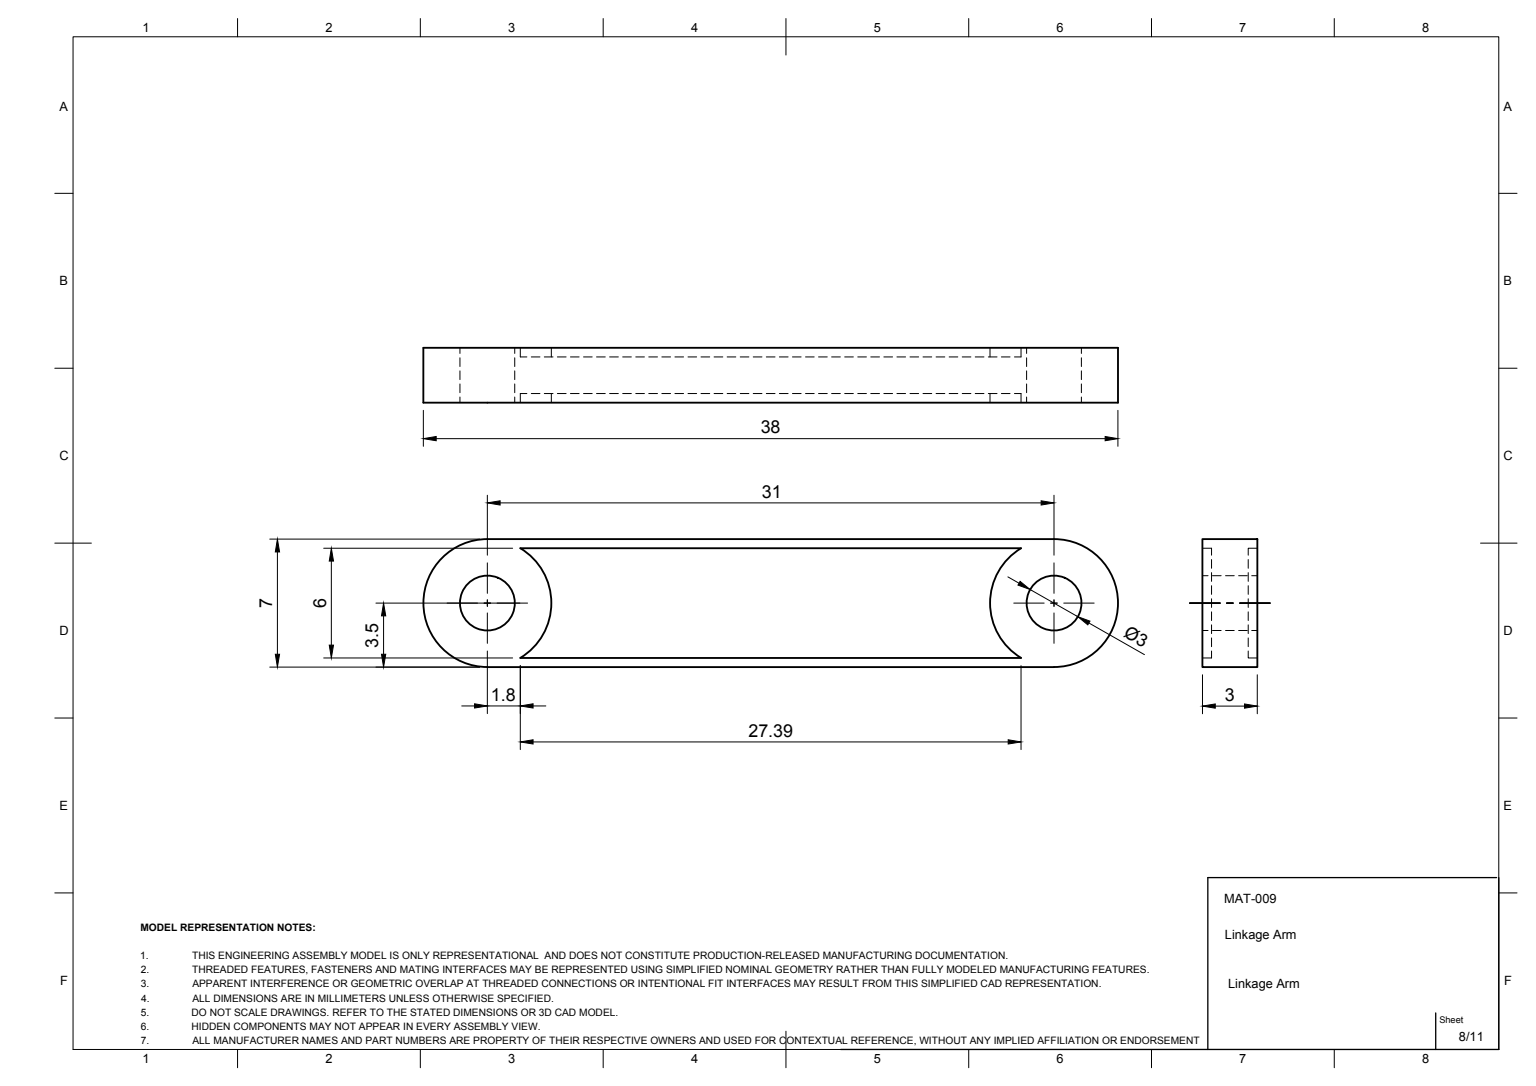
ISO-10303-21;
HEADER;
/* Generated by software containing ST-Developer
 * from STEP Tools, Inc. (www.steptools.com) 
 */

FILE_DESCRIPTION(
/* description */ ('STEP AP214'),
/* implementation_level */ '2;1');

FILE_NAME(
/* name */ 'Linkage Arm.step',
/* time_stamp */ '2026-11-14T05:43:09-08:00',
/* author */ (''),
/* organization */ (''),
/* preprocessor_version */ 'ST-DEVELOPER v20.2',
/* originating_system */ 'Autodesk Translation Framework v15.17.0.0',
/* authorisation */ '');

FILE_SCHEMA (('AUTOMOTIVE_DESIGN { 1 0 10303 214 3 1 1 }'));
ENDSEC;

DATA;
#10=MECHANICAL_DESIGN_GEOMETRIC_PRESENTATION_REPRESENTATION('',(#152),#11933);
#134=SHAPE_REPRESENTATION_RELATIONSHIP('SRR','None',#11994,#143);
#143=ADVANCED_BREP_SHAPE_REPRESENTATION('',(#161),#11930);
#152=STYLED_ITEM('',(#12044),#161);
#161=MANIFOLD_SOLID_BREP('Body1',#6649);
#200=FACE_BOUND('',#1019,.T.);
#201=FACE_BOUND('',#1020,.T.);
#202=FACE_BOUND('',#1021,.T.);
#203=FACE_BOUND('',#1026,.T.);
#204=FACE_BOUND('',#1027,.T.);
#205=FACE_BOUND('',#1028,.T.);
#288=PLANE('',#7537);
#289=PLANE('',#7540);
#290=PLANE('',#7541);
#291=PLANE('',#7544);
#292=PLANE('',#7546);
#293=PLANE('',#7549);
#294=PLANE('',#7550);
#295=PLANE('',#7553);
#296=PLANE('',#7554);
#297=PLANE('',#7555);
#623=FACE_OUTER_BOUND('',#1013,.T.);
#624=FACE_OUTER_BOUND('',#1014,.T.);
#625=FACE_OUTER_BOUND('',#1015,.T.);
#626=FACE_OUTER_BOUND('',#1016,.T.);
#627=FACE_OUTER_BOUND('',#1017,.T.);
#628=FACE_OUTER_BOUND('',#1018,.T.);
#629=FACE_OUTER_BOUND('',#1022,.T.);
#630=FACE_OUTER_BOUND('',#1023,.T.);
#631=FACE_OUTER_BOUND('',#1024,.T.);
#632=FACE_OUTER_BOUND('',#1025,.T.);
#633=FACE_OUTER_BOUND('',#1029,.T.);
#634=FACE_OUTER_BOUND('',#1030,.T.);
#635=FACE_OUTER_BOUND('',#1031,.T.);
#636=FACE_OUTER_BOUND('',#1032,.T.);
#637=FACE_OUTER_BOUND('',#1033,.T.);
#638=FACE_OUTER_BOUND('',#1034,.T.);
#639=FACE_OUTER_BOUND('',#1035,.T.);
#640=FACE_OUTER_BOUND('',#1036,.T.);
#1013=EDGE_LOOP('',(#5812,#5813,#5814,#5815));
#1014=EDGE_LOOP('',(#5816,#5817,#5818,#5819));
#1015=EDGE_LOOP('',(#5820,#5821,#5822,#5823));
#1016=EDGE_LOOP('',(#5824,#5825,#5826,#5827));
#1017=EDGE_LOOP('',(#5828,#5829,#5830,#5831));
#1018=EDGE_LOOP('',(#5832,#5833,#5834,#5835));
#1019=EDGE_LOOP('',(#5836));
#1020=EDGE_LOOP('',(#5837));
#1021=EDGE_LOOP('',(#5838,#5839,#5840,#5841));
#1022=EDGE_LOOP('',(#5842,#5843,#5844,#5845));
#1023=EDGE_LOOP('',(#5846,#5847,#5848,#5849));
#1024=EDGE_LOOP('',(#5850,#5851,#5852,#5853));
#1025=EDGE_LOOP('',(#5854,#5855,#5856,#5857));
#1026=EDGE_LOOP('',(#5858,#5859,#5860,#5861));
#1027=EDGE_LOOP('',(#5862));
#1028=EDGE_LOOP('',(#5863));
#1029=EDGE_LOOP('',(#5864,#5865,#5866,#5867));
#1030=EDGE_LOOP('',(#5868,#5869,#5870,#5871));
#1031=EDGE_LOOP('',(#5872,#5873,#5874,#5875));
#1032=EDGE_LOOP('',(#5876,#5877,#5878,#5879));
#1033=EDGE_LOOP('',(#5880,#5881,#5882,#5883));
#1034=EDGE_LOOP('',(#5884,#5885,#5886,#5887));
#1035=EDGE_LOOP('',(#5888,#5889,#5890,#5891));
#1036=EDGE_LOOP('',(#5892,#5893,#5894,#5895));
#1464=LINE('',#11641,#1926);
#1465=LINE('',#11644,#1927);
#1466=LINE('',#11650,#1928);
#1467=LINE('',#11653,#1929);
#1468=LINE('',#11658,#1930);
#1469=LINE('',#11664,#1931);
#1470=LINE('',#11671,#1932);
#1471=LINE('',#11674,#1933);
#1472=LINE('',#11677,#1934);
#1473=LINE('',#11680,#1935);
#1474=LINE('',#11684,#1936);
#1475=LINE('',#11685,#1937);
#1476=LINE('',#11688,#1938);
#1477=LINE('',#11689,#1939);
#1478=LINE('',#11692,#1940);
#1479=LINE('',#11693,#1941);
#1480=LINE('',#11698,#1942);
#1481=LINE('',#11701,#1943);
#1482=LINE('',#11704,#1944);
#1483=LINE('',#11705,#1945);
#1484=LINE('',#11709,#1946);
#1485=LINE('',#11711,#1947);
#1486=LINE('',#11715,#1948);
#1487=LINE('',#11718,#1949);
#1488=LINE('',#11720,#1950);
#1489=LINE('',#11722,#1951);
#1926=VECTOR('',#9586,1000.);
#1927=VECTOR('',#9589,1000.);
#1928=VECTOR('',#9594,1000.);
#1929=VECTOR('',#9597,1000.);
#1930=VECTOR('',#9602,1.5);
#1931=VECTOR('',#9609,1.5);
#1932=VECTOR('',#9616,1000.);
#1933=VECTOR('',#9619,1000.);
#1934=VECTOR('',#9622,1000.);
#1935=VECTOR('',#9625,1000.);
#1936=VECTOR('',#9628,1000.);
#1937=VECTOR('',#9629,1000.);
#1938=VECTOR('',#9632,1000.);
#1939=VECTOR('',#9633,1000.);
#1940=VECTOR('',#9636,1000.);
#1941=VECTOR('',#9637,1000.);
#1942=VECTOR('',#9644,1000.);
#1943=VECTOR('',#9647,1000.);
#1944=VECTOR('',#9650,1000.);
#1945=VECTOR('',#9651,1000.);
#1946=VECTOR('',#9656,1000.);
#1947=VECTOR('',#9659,1000.);
#1948=VECTOR('',#9664,1000.);
#1949=VECTOR('',#9667,1000.);
#1950=VECTOR('',#9670,1000.);
#1951=VECTOR('',#9673,1000.);
#2454=CIRCLE('',#7523,3.5);
#2455=CIRCLE('',#7524,3.5);
#2456=CIRCLE('',#7526,3.5);
#2457=CIRCLE('',#7527,3.5);
#2458=CIRCLE('',#7529,1.5);
#2459=CIRCLE('',#7530,1.5);
#2460=CIRCLE('',#7532,1.5);
#2461=CIRCLE('',#7533,1.5);
#2462=CIRCLE('',#7535,3.5);
#2463=CIRCLE('',#7536,3.5);
#2464=CIRCLE('',#7538,3.5);
#2465=CIRCLE('',#7539,3.5);
#2466=CIRCLE('',#7543,3.5);
#2467=CIRCLE('',#7545,3.5);
#2468=CIRCLE('',#7548,3.5);
#2469=CIRCLE('',#7552,3.5);
#3067=VERTEX_POINT('',#11637);
#3068=VERTEX_POINT('',#11638);
#3069=VERTEX_POINT('',#11640);
#3070=VERTEX_POINT('',#11642);
#3071=VERTEX_POINT('',#11646);
#3072=VERTEX_POINT('',#11647);
#3073=VERTEX_POINT('',#11649);
#3074=VERTEX_POINT('',#11651);
#3075=VERTEX_POINT('',#11655);
#3076=VERTEX_POINT('',#11657);
#3077=VERTEX_POINT('',#11661);
#3078=VERTEX_POINT('',#11663);
#3079=VERTEX_POINT('',#11667);
#3080=VERTEX_POINT('',#11668);
#3081=VERTEX_POINT('',#11670);
#3082=VERTEX_POINT('',#11672);
#3083=VERTEX_POINT('',#11676);
#3084=VERTEX_POINT('',#11678);
#3085=VERTEX_POINT('',#11681);
#3086=VERTEX_POINT('',#11682);
#3087=VERTEX_POINT('',#11687);
#3088=VERTEX_POINT('',#11691);
#3089=VERTEX_POINT('',#11697);
#3090=VERTEX_POINT('',#11699);
#3091=VERTEX_POINT('',#11703);
#3092=VERTEX_POINT('',#11707);
#3093=VERTEX_POINT('',#11714);
#3094=VERTEX_POINT('',#11716);
#3995=EDGE_CURVE('',#3067,#3068,#2454,.T.);
#3996=EDGE_CURVE('',#3068,#3069,#1464,.T.);
#3997=EDGE_CURVE('',#3070,#3069,#2455,.T.);
#3998=EDGE_CURVE('',#3067,#3070,#1465,.T.);
#3999=EDGE_CURVE('',#3071,#3072,#2456,.T.);
#4000=EDGE_CURVE('',#3071,#3073,#1466,.T.);
#4001=EDGE_CURVE('',#3073,#3074,#2457,.T.);
#4002=EDGE_CURVE('',#3072,#3074,#1467,.T.);
#4003=EDGE_CURVE('',#3075,#3075,#2458,.T.);
#4004=EDGE_CURVE('',#3075,#3076,#1468,.T.);
#4005=EDGE_CURVE('',#3076,#3076,#2459,.T.);
#4006=EDGE_CURVE('',#3077,#3077,#2460,.T.);
#4007=EDGE_CURVE('',#3077,#3078,#1469,.T.);
#4008=EDGE_CURVE('',#3078,#3078,#2461,.T.);
#4009=EDGE_CURVE('',#3079,#3080,#2462,.T.);
#4010=EDGE_CURVE('',#3079,#3081,#1470,.T.);
#4011=EDGE_CURVE('',#3081,#3082,#2463,.T.);
#4012=EDGE_CURVE('',#3080,#3082,#1471,.T.);
#4013=EDGE_CURVE('',#3083,#3081,#1472,.T.);
#4014=EDGE_CURVE('',#3084,#3083,#2464,.T.);
#4015=EDGE_CURVE('',#3082,#3084,#1473,.T.);
#4016=EDGE_CURVE('',#3085,#3086,#2465,.T.);
#4017=EDGE_CURVE('',#3086,#3070,#1474,.T.);
#4018=EDGE_CURVE('',#3069,#3085,#1475,.T.);
#4019=EDGE_CURVE('',#3087,#3079,#1476,.T.);
#4020=EDGE_CURVE('',#3087,#3083,#1477,.T.);
#4021=EDGE_CURVE('',#3088,#3084,#1478,.T.);
#4022=EDGE_CURVE('',#3080,#3088,#1479,.T.);
#4023=EDGE_CURVE('',#3088,#3087,#2466,.T.);
#4024=EDGE_CURVE('',#3089,#3073,#1480,.T.);
#4025=EDGE_CURVE('',#3090,#3089,#2467,.T.);
#4026=EDGE_CURVE('',#3074,#3090,#1481,.T.);
#4027=EDGE_CURVE('',#3091,#3071,#1482,.T.);
#4028=EDGE_CURVE('',#3091,#3089,#1483,.T.);
#4029=EDGE_CURVE('',#3092,#3091,#2468,.T.);
#4030=EDGE_CURVE('',#3092,#3090,#1484,.T.);
#4031=EDGE_CURVE('',#3072,#3092,#1485,.T.);
#4032=EDGE_CURVE('',#3093,#3085,#1486,.T.);
#4033=EDGE_CURVE('',#3093,#3094,#2469,.T.);
#4034=EDGE_CURVE('',#3094,#3086,#1487,.T.);
#4035=EDGE_CURVE('',#3094,#3067,#1488,.T.);
#4036=EDGE_CURVE('',#3068,#3093,#1489,.T.);
#5812=ORIENTED_EDGE('',*,*,#3995,.T.);
#5813=ORIENTED_EDGE('',*,*,#3996,.T.);
#5814=ORIENTED_EDGE('',*,*,#3997,.F.);
#5815=ORIENTED_EDGE('',*,*,#3998,.F.);
#5816=ORIENTED_EDGE('',*,*,#3999,.F.);
#5817=ORIENTED_EDGE('',*,*,#4000,.T.);
#5818=ORIENTED_EDGE('',*,*,#4001,.T.);
#5819=ORIENTED_EDGE('',*,*,#4002,.F.);
#5820=ORIENTED_EDGE('',*,*,#4003,.T.);
#5821=ORIENTED_EDGE('',*,*,#4004,.T.);
#5822=ORIENTED_EDGE('',*,*,#4005,.F.);
#5823=ORIENTED_EDGE('',*,*,#4004,.F.);
#5824=ORIENTED_EDGE('',*,*,#4006,.T.);
#5825=ORIENTED_EDGE('',*,*,#4007,.T.);
#5826=ORIENTED_EDGE('',*,*,#4008,.F.);
#5827=ORIENTED_EDGE('',*,*,#4007,.F.);
#5828=ORIENTED_EDGE('',*,*,#4009,.F.);
#5829=ORIENTED_EDGE('',*,*,#4010,.T.);
#5830=ORIENTED_EDGE('',*,*,#4011,.T.);
#5831=ORIENTED_EDGE('',*,*,#4012,.F.);
#5832=ORIENTED_EDGE('',*,*,#4013,.F.);
#5833=ORIENTED_EDGE('',*,*,#4014,.F.);
#5834=ORIENTED_EDGE('',*,*,#4015,.F.);
#5835=ORIENTED_EDGE('',*,*,#4011,.F.);
#5836=ORIENTED_EDGE('',*,*,#4008,.T.);
#5837=ORIENTED_EDGE('',*,*,#4005,.T.);
#5838=ORIENTED_EDGE('',*,*,#4016,.T.);
#5839=ORIENTED_EDGE('',*,*,#4017,.T.);
#5840=ORIENTED_EDGE('',*,*,#3997,.T.);
#5841=ORIENTED_EDGE('',*,*,#4018,.T.);
#5842=ORIENTED_EDGE('',*,*,#4013,.T.);
#5843=ORIENTED_EDGE('',*,*,#4010,.F.);
#5844=ORIENTED_EDGE('',*,*,#4019,.F.);
#5845=ORIENTED_EDGE('',*,*,#4020,.T.);
#5846=ORIENTED_EDGE('',*,*,#4015,.T.);
#5847=ORIENTED_EDGE('',*,*,#4021,.F.);
#5848=ORIENTED_EDGE('',*,*,#4022,.F.);
#5849=ORIENTED_EDGE('',*,*,#4012,.T.);
#5850=ORIENTED_EDGE('',*,*,#4014,.T.);
#5851=ORIENTED_EDGE('',*,*,#4020,.F.);
#5852=ORIENTED_EDGE('',*,*,#4023,.F.);
#5853=ORIENTED_EDGE('',*,*,#4021,.T.);
#5854=ORIENTED_EDGE('',*,*,#4019,.T.);
#5855=ORIENTED_EDGE('',*,*,#4009,.T.);
#5856=ORIENTED_EDGE('',*,*,#4022,.T.);
#5857=ORIENTED_EDGE('',*,*,#4023,.T.);
#5858=ORIENTED_EDGE('',*,*,#4001,.F.);
#5859=ORIENTED_EDGE('',*,*,#4024,.F.);
#5860=ORIENTED_EDGE('',*,*,#4025,.F.);
#5861=ORIENTED_EDGE('',*,*,#4026,.F.);
#5862=ORIENTED_EDGE('',*,*,#4003,.F.);
#5863=ORIENTED_EDGE('',*,*,#4006,.F.);
#5864=ORIENTED_EDGE('',*,*,#4024,.T.);
#5865=ORIENTED_EDGE('',*,*,#4000,.F.);
#5866=ORIENTED_EDGE('',*,*,#4027,.F.);
#5867=ORIENTED_EDGE('',*,*,#4028,.T.);
#5868=ORIENTED_EDGE('',*,*,#4025,.T.);
#5869=ORIENTED_EDGE('',*,*,#4028,.F.);
#5870=ORIENTED_EDGE('',*,*,#4029,.F.);
#5871=ORIENTED_EDGE('',*,*,#4030,.T.);
#5872=ORIENTED_EDGE('',*,*,#4026,.T.);
#5873=ORIENTED_EDGE('',*,*,#4030,.F.);
#5874=ORIENTED_EDGE('',*,*,#4031,.F.);
#5875=ORIENTED_EDGE('',*,*,#4002,.T.);
#5876=ORIENTED_EDGE('',*,*,#3999,.T.);
#5877=ORIENTED_EDGE('',*,*,#4031,.T.);
#5878=ORIENTED_EDGE('',*,*,#4029,.T.);
#5879=ORIENTED_EDGE('',*,*,#4027,.T.);
#5880=ORIENTED_EDGE('',*,*,#4016,.F.);
#5881=ORIENTED_EDGE('',*,*,#4032,.F.);
#5882=ORIENTED_EDGE('',*,*,#4033,.T.);
#5883=ORIENTED_EDGE('',*,*,#4034,.T.);
#5884=ORIENTED_EDGE('',*,*,#4017,.F.);
#5885=ORIENTED_EDGE('',*,*,#4034,.F.);
#5886=ORIENTED_EDGE('',*,*,#4035,.T.);
#5887=ORIENTED_EDGE('',*,*,#3998,.T.);
#5888=ORIENTED_EDGE('',*,*,#4018,.F.);
#5889=ORIENTED_EDGE('',*,*,#3996,.F.);
#5890=ORIENTED_EDGE('',*,*,#4036,.T.);
#5891=ORIENTED_EDGE('',*,*,#4032,.T.);
#5892=ORIENTED_EDGE('',*,*,#4033,.F.);
#5893=ORIENTED_EDGE('',*,*,#4036,.F.);
#5894=ORIENTED_EDGE('',*,*,#3995,.F.);
#5895=ORIENTED_EDGE('',*,*,#4035,.F.);
#6271=CYLINDRICAL_SURFACE('',#7522,3.5);
#6272=CYLINDRICAL_SURFACE('',#7525,3.5);
#6273=CYLINDRICAL_SURFACE('',#7528,1.5);
#6274=CYLINDRICAL_SURFACE('',#7531,1.5);
#6275=CYLINDRICAL_SURFACE('',#7534,3.5);
#6276=CYLINDRICAL_SURFACE('',#7542,3.5);
#6277=CYLINDRICAL_SURFACE('',#7547,3.5);
#6278=CYLINDRICAL_SURFACE('',#7551,3.5);
#6593=ADVANCED_FACE('',(#623),#6271,.T.);
#6594=ADVANCED_FACE('',(#624),#6272,.T.);
#6595=ADVANCED_FACE('',(#625),#6273,.F.);
#6596=ADVANCED_FACE('',(#626),#6274,.F.);
#6597=ADVANCED_FACE('',(#627),#6275,.T.);
#6598=ADVANCED_FACE('',(#628,#200,#201,#202),#288,.F.);
#6599=ADVANCED_FACE('',(#629),#289,.F.);
#6600=ADVANCED_FACE('',(#630),#290,.F.);
#6601=ADVANCED_FACE('',(#631),#6276,.T.);
#6602=ADVANCED_FACE('',(#632,#203,#204,#205),#291,.T.);
#6603=ADVANCED_FACE('',(#633),#292,.F.);
#6604=ADVANCED_FACE('',(#634),#6277,.T.);
#6605=ADVANCED_FACE('',(#635),#293,.F.);
#6606=ADVANCED_FACE('',(#636),#294,.T.);
#6607=ADVANCED_FACE('',(#637),#6278,.T.);
#6608=ADVANCED_FACE('',(#638),#295,.T.);
#6609=ADVANCED_FACE('',(#639),#296,.T.);
#6610=ADVANCED_FACE('',(#640),#297,.T.);
#6649=CLOSED_SHELL('',(#6593,#6594,#6595,#6596,#6597,#6598,#6599,#6600,
#6601,#6602,#6603,#6604,#6605,#6606,#6607,#6608,#6609,#6610));
#7521=AXIS2_PLACEMENT_3D('',#11635,#9580,#9581);
#7522=AXIS2_PLACEMENT_3D('',#11636,#9582,#9583);
#7523=AXIS2_PLACEMENT_3D('',#11639,#9584,#9585);
#7524=AXIS2_PLACEMENT_3D('',#11643,#9587,#9588);
#7525=AXIS2_PLACEMENT_3D('',#11645,#9590,#9591);
#7526=AXIS2_PLACEMENT_3D('',#11648,#9592,#9593);
#7527=AXIS2_PLACEMENT_3D('',#11652,#9595,#9596);
#7528=AXIS2_PLACEMENT_3D('',#11654,#9598,#9599);
#7529=AXIS2_PLACEMENT_3D('',#11656,#9600,#9601);
#7530=AXIS2_PLACEMENT_3D('',#11659,#9603,#9604);
#7531=AXIS2_PLACEMENT_3D('',#11660,#9605,#9606);
#7532=AXIS2_PLACEMENT_3D('',#11662,#9607,#9608);
#7533=AXIS2_PLACEMENT_3D('',#11665,#9610,#9611);
#7534=AXIS2_PLACEMENT_3D('',#11666,#9612,#9613);
#7535=AXIS2_PLACEMENT_3D('',#11669,#9614,#9615);
#7536=AXIS2_PLACEMENT_3D('',#11673,#9617,#9618);
#7537=AXIS2_PLACEMENT_3D('',#11675,#9620,#9621);
#7538=AXIS2_PLACEMENT_3D('',#11679,#9623,#9624);
#7539=AXIS2_PLACEMENT_3D('',#11683,#9626,#9627);
#7540=AXIS2_PLACEMENT_3D('',#11686,#9630,#9631);
#7541=AXIS2_PLACEMENT_3D('',#11690,#9634,#9635);
#7542=AXIS2_PLACEMENT_3D('',#11694,#9638,#9639);
#7543=AXIS2_PLACEMENT_3D('',#11695,#9640,#9641);
#7544=AXIS2_PLACEMENT_3D('',#11696,#9642,#9643);
#7545=AXIS2_PLACEMENT_3D('',#11700,#9645,#9646);
#7546=AXIS2_PLACEMENT_3D('',#11702,#9648,#9649);
#7547=AXIS2_PLACEMENT_3D('',#11706,#9652,#9653);
#7548=AXIS2_PLACEMENT_3D('',#11708,#9654,#9655);
#7549=AXIS2_PLACEMENT_3D('',#11710,#9657,#9658);
#7550=AXIS2_PLACEMENT_3D('',#11712,#9660,#9661);
#7551=AXIS2_PLACEMENT_3D('',#11713,#9662,#9663);
#7552=AXIS2_PLACEMENT_3D('',#11717,#9665,#9666);
#7553=AXIS2_PLACEMENT_3D('',#11719,#9668,#9669);
#7554=AXIS2_PLACEMENT_3D('',#11721,#9671,#9672);
#7555=AXIS2_PLACEMENT_3D('',#11723,#9674,#9675);
#9580=DIRECTION('axis',(0.,0.,1.));
#9581=DIRECTION('refdir',(1.,0.,0.));
#9582=DIRECTION('center_axis',(0.,0.,-1.));
#9583=DIRECTION('ref_axis',(-1.,0.,0.));
#9584=DIRECTION('center_axis',(0.,0.,-1.));
#9585=DIRECTION('ref_axis',(1.,0.,0.));
#9586=DIRECTION('',(0.,0.,-1.));
#9587=DIRECTION('center_axis',(0.,0.,-1.));
#9588=DIRECTION('ref_axis',(1.,0.,0.));
#9589=DIRECTION('',(0.,0.,-1.));
#9590=DIRECTION('center_axis',(0.,0.,1.));
#9591=DIRECTION('ref_axis',(1.,0.,0.));
#9592=DIRECTION('center_axis',(0.,0.,-1.));
#9593=DIRECTION('ref_axis',(1.,0.,0.));
#9594=DIRECTION('',(0.,0.,1.));
#9595=DIRECTION('center_axis',(0.,0.,-1.));
#9596=DIRECTION('ref_axis',(1.,0.,0.));
#9597=DIRECTION('',(0.,0.,1.));
#9598=DIRECTION('center_axis',(0.,0.,-1.));
#9599=DIRECTION('ref_axis',(-1.,0.,0.));
#9600=DIRECTION('center_axis',(0.,0.,1.));
#9601=DIRECTION('ref_axis',(1.,0.,0.));
#9602=DIRECTION('',(0.,0.,-1.));
#9603=DIRECTION('center_axis',(0.,0.,1.));
#9604=DIRECTION('ref_axis',(1.,0.,0.));
#9605=DIRECTION('center_axis',(0.,0.,-1.));
#9606=DIRECTION('ref_axis',(-1.,0.,0.));
#9607=DIRECTION('center_axis',(0.,0.,1.));
#9608=DIRECTION('ref_axis',(1.,0.,0.));
#9609=DIRECTION('',(0.,0.,-1.));
#9610=DIRECTION('center_axis',(0.,0.,1.));
#9611=DIRECTION('ref_axis',(1.,0.,0.));
#9612=DIRECTION('center_axis',(0.,0.,-1.));
#9613=DIRECTION('ref_axis',(-1.,0.,0.));
#9614=DIRECTION('center_axis',(0.,0.,1.));
#9615=DIRECTION('ref_axis',(1.,0.,0.));
#9616=DIRECTION('',(0.,0.,-1.));
#9617=DIRECTION('center_axis',(0.,0.,1.));
#9618=DIRECTION('ref_axis',(1.,0.,0.));
#9619=DIRECTION('',(0.,0.,-1.));
#9620=DIRECTION('center_axis',(0.,0.,1.));
#9621=DIRECTION('ref_axis',(1.,0.,0.));
#9622=DIRECTION('',(-1.,0.,0.));
#9623=DIRECTION('center_axis',(0.,0.,1.));
#9624=DIRECTION('ref_axis',(1.,0.,0.));
#9625=DIRECTION('',(1.,0.,0.));
#9626=DIRECTION('center_axis',(0.,0.,-1.));
#9627=DIRECTION('ref_axis',(1.,0.,0.));
#9628=DIRECTION('',(1.,-3.16619526353726E-17,0.));
#9629=DIRECTION('',(-1.,3.16619526353726E-17,0.));
#9630=DIRECTION('center_axis',(0.,-1.,0.));
#9631=DIRECTION('ref_axis',(0.,0.,-1.));
#9632=DIRECTION('',(-1.,0.,0.));
#9633=DIRECTION('',(0.,0.,-1.));
#9634=DIRECTION('center_axis',(0.,1.,0.));
#9635=DIRECTION('ref_axis',(0.,0.,1.));
#9636=DIRECTION('',(0.,0.,-1.));
#9637=DIRECTION('',(1.,0.,0.));
#9638=DIRECTION('center_axis',(0.,0.,-1.));
#9639=DIRECTION('ref_axis',(1.,1.22464679914735E-16,0.));
#9640=DIRECTION('center_axis',(0.,0.,1.));
#9641=DIRECTION('ref_axis',(1.,0.,0.));
#9642=DIRECTION('center_axis',(0.,0.,1.));
#9643=DIRECTION('ref_axis',(1.,0.,0.));
#9644=DIRECTION('',(-1.,3.16619526353726E-17,0.));
#9645=DIRECTION('center_axis',(0.,0.,-1.));
#9646=DIRECTION('ref_axis',(1.,0.,0.));
#9647=DIRECTION('',(1.,-3.16619526353726E-17,0.));
#9648=DIRECTION('center_axis',(3.16619526353726E-17,1.,0.));
#9649=DIRECTION('ref_axis',(-1.,3.16619526353726E-17,0.));
#9650=DIRECTION('',(-1.,3.16619526353726E-17,0.));
#9651=DIRECTION('',(0.,0.,1.));
#9652=DIRECTION('center_axis',(0.,0.,1.));
#9653=DIRECTION('ref_axis',(-1.,1.22464679914735E-16,0.));
#9654=DIRECTION('center_axis',(0.,0.,-1.));
#9655=DIRECTION('ref_axis',(1.,0.,0.));
#9656=DIRECTION('',(0.,0.,1.));
#9657=DIRECTION('center_axis',(-3.16619526353726E-17,-1.,0.));
#9658=DIRECTION('ref_axis',(1.,-3.16619526353726E-17,0.));
#9659=DIRECTION('',(1.,-3.16619526353726E-17,0.));
#9660=DIRECTION('center_axis',(0.,0.,1.));
#9661=DIRECTION('ref_axis',(1.,0.,0.));
#9662=DIRECTION('center_axis',(0.,0.,-1.));
#9663=DIRECTION('ref_axis',(1.,5.66553889764798E-16,0.));
#9664=DIRECTION('',(0.,0.,-1.));
#9665=DIRECTION('center_axis',(0.,0.,-1.));
#9666=DIRECTION('ref_axis',(1.,0.,0.));
#9667=DIRECTION('',(0.,0.,-1.));
#9668=DIRECTION('center_axis',(3.16619526353726E-17,1.,0.));
#9669=DIRECTION('ref_axis',(-1.,3.16619526353726E-17,0.));
#9670=DIRECTION('',(1.,-3.16619526353726E-17,0.));
#9671=DIRECTION('center_axis',(-3.16619526353726E-17,-1.,0.));
#9672=DIRECTION('ref_axis',(1.,-3.16619526353726E-17,0.));
#9673=DIRECTION('',(-1.,3.16619526353726E-17,0.));
#9674=DIRECTION('center_axis',(0.,0.,-1.));
#9675=DIRECTION('ref_axis',(1.,0.,0.));
#11635=CARTESIAN_POINT('',(0.,0.,0.));
#11636=CARTESIAN_POINT('Origin',(31.,3.5,0.5));
#11637=CARTESIAN_POINT('',(29.197224362268,0.5,0.5));
#11638=CARTESIAN_POINT('',(29.197224362268,6.5,0.5));
#11639=CARTESIAN_POINT('Origin',(31.,3.5,0.5));
#11640=CARTESIAN_POINT('',(29.197224362268,6.5,0.));
#11641=CARTESIAN_POINT('',(29.197224362268,6.5,0.5));
#11642=CARTESIAN_POINT('',(29.197224362268,0.5,0.));
#11643=CARTESIAN_POINT('Origin',(31.,3.5,0.));
#11644=CARTESIAN_POINT('',(29.197224362268,0.5,0.5));
#11645=CARTESIAN_POINT('Origin',(0.,3.5,2.5));
#11646=CARTESIAN_POINT('',(1.80277563773199,6.5,2.5));
#11647=CARTESIAN_POINT('',(1.802775637732,0.500000000000001,2.5));
#11648=CARTESIAN_POINT('Origin',(0.,3.5,2.5));
#11649=CARTESIAN_POINT('',(1.80277563773199,6.5,3.));
#11650=CARTESIAN_POINT('',(1.80277563773199,6.5,2.5));
#11651=CARTESIAN_POINT('',(1.802775637732,0.500000000000001,3.));
#11652=CARTESIAN_POINT('Origin',(0.,3.5,3.));
#11653=CARTESIAN_POINT('',(1.802775637732,0.500000000000001,2.5));
#11654=CARTESIAN_POINT('Origin',(31.,3.5,3.));
#11655=CARTESIAN_POINT('',(32.5,3.5,3.));
#11656=CARTESIAN_POINT('Origin',(31.,3.5,3.));
#11657=CARTESIAN_POINT('',(32.5,3.5,0.));
#11658=CARTESIAN_POINT('',(32.5,3.5,3.));
#11659=CARTESIAN_POINT('Origin',(31.,3.5,0.));
#11660=CARTESIAN_POINT('Origin',(0.,3.5,3.));
#11661=CARTESIAN_POINT('',(1.5,3.5,3.));
#11662=CARTESIAN_POINT('Origin',(0.,3.5,3.));
#11663=CARTESIAN_POINT('',(1.5,3.5,0.));
#11664=CARTESIAN_POINT('',(1.5,3.5,3.));
#11665=CARTESIAN_POINT('Origin',(0.,3.5,0.));
#11666=CARTESIAN_POINT('Origin',(0.,3.5,3.));
#11667=CARTESIAN_POINT('',(0.,7.,3.));
#11668=CARTESIAN_POINT('',(0.,0.,3.));
#11669=CARTESIAN_POINT('Origin',(0.,3.5,3.));
#11670=CARTESIAN_POINT('',(0.,7.,0.));
#11671=CARTESIAN_POINT('',(0.,7.,3.));
#11672=CARTESIAN_POINT('',(0.,0.,0.));
#11673=CARTESIAN_POINT('Origin',(0.,3.5,0.));
#11674=CARTESIAN_POINT('',(0.,0.,3.));
#11675=CARTESIAN_POINT('Origin',(0.,0.,0.));
#11676=CARTESIAN_POINT('',(31.,7.,0.));
#11677=CARTESIAN_POINT('',(0.,7.,0.));
#11678=CARTESIAN_POINT('',(31.,0.,0.));
#11679=CARTESIAN_POINT('Origin',(31.,3.5,0.));
#11680=CARTESIAN_POINT('',(0.,0.,0.));
#11681=CARTESIAN_POINT('',(1.80277563773199,6.5,0.));
#11682=CARTESIAN_POINT('',(1.802775637732,0.500000000000001,0.));
#11683=CARTESIAN_POINT('Origin',(0.,3.5,0.));
#11684=CARTESIAN_POINT('',(1.802775637732,0.500000000000001,0.));
#11685=CARTESIAN_POINT('',(1.80277563773199,6.5,0.));
#11686=CARTESIAN_POINT('Origin',(0.,7.,3.));
#11687=CARTESIAN_POINT('',(31.,7.,3.));
#11688=CARTESIAN_POINT('',(0.,7.,3.));
#11689=CARTESIAN_POINT('',(31.,7.,3.));
#11690=CARTESIAN_POINT('Origin',(0.,0.,3.));
#11691=CARTESIAN_POINT('',(31.,0.,3.));
#11692=CARTESIAN_POINT('',(31.,0.,3.));
#11693=CARTESIAN_POINT('',(0.,0.,3.));
#11694=CARTESIAN_POINT('Origin',(31.,3.5,3.));
#11695=CARTESIAN_POINT('Origin',(31.,3.5,3.));
#11696=CARTESIAN_POINT('Origin',(0.,0.,3.));
#11697=CARTESIAN_POINT('',(29.197224362268,6.5,3.));
#11698=CARTESIAN_POINT('',(1.80277563773199,6.5,3.));
#11699=CARTESIAN_POINT('',(29.197224362268,0.5,3.));
#11700=CARTESIAN_POINT('Origin',(31.,3.5,3.));
#11701=CARTESIAN_POINT('',(1.802775637732,0.500000000000001,3.));
#11702=CARTESIAN_POINT('Origin',(1.80277563773199,6.5,2.5));
#11703=CARTESIAN_POINT('',(29.197224362268,6.5,2.5));
#11704=CARTESIAN_POINT('',(1.80277563773199,6.5,2.5));
#11705=CARTESIAN_POINT('',(29.197224362268,6.5,2.5));
#11706=CARTESIAN_POINT('Origin',(31.,3.5,2.5));
#11707=CARTESIAN_POINT('',(29.197224362268,0.5,2.5));
#11708=CARTESIAN_POINT('Origin',(31.,3.5,2.5));
#11709=CARTESIAN_POINT('',(29.197224362268,0.5,2.5));
#11710=CARTESIAN_POINT('Origin',(1.802775637732,0.500000000000001,2.5));
#11711=CARTESIAN_POINT('',(1.802775637732,0.500000000000001,2.5));
#11712=CARTESIAN_POINT('Origin',(0.,3.5,2.5));
#11713=CARTESIAN_POINT('Origin',(0.,3.5,0.5));
#11714=CARTESIAN_POINT('',(1.80277563773199,6.5,0.5));
#11715=CARTESIAN_POINT('',(1.80277563773199,6.5,0.5));
#11716=CARTESIAN_POINT('',(1.802775637732,0.500000000000001,0.5));
#11717=CARTESIAN_POINT('Origin',(0.,3.5,0.5));
#11718=CARTESIAN_POINT('',(1.802775637732,0.500000000000001,0.5));
#11719=CARTESIAN_POINT('Origin',(1.802775637732,0.500000000000001,0.5));
#11720=CARTESIAN_POINT('',(1.802775637732,0.500000000000001,0.5));
#11721=CARTESIAN_POINT('Origin',(1.80277563773199,6.5,0.5));
#11722=CARTESIAN_POINT('',(1.80277563773199,6.5,0.5));
#11723=CARTESIAN_POINT('Origin',(0.,3.5,0.5));
#11919=UNCERTAINTY_MEASURE_WITH_UNIT(LENGTH_MEASURE(0.01),#11934,
'DISTANCE_ACCURACY_VALUE',
'Maximum model space distance between geometric entities at asserted c
onnectivities');
#11922=UNCERTAINTY_MEASURE_WITH_UNIT(LENGTH_MEASURE(0.01),#11934,
'DISTANCE_ACCURACY_VALUE',
'Maximum model space distance between geometric entities at asserted c
onnectivities');
#11930=(
GEOMETRIC_REPRESENTATION_CONTEXT(3)
GLOBAL_UNCERTAINTY_ASSIGNED_CONTEXT((#11919))
GLOBAL_UNIT_ASSIGNED_CONTEXT((#11934,#11936,#11937))
REPRESENTATION_CONTEXT('','3D')
);
#11933=(
GEOMETRIC_REPRESENTATION_CONTEXT(3)
GLOBAL_UNCERTAINTY_ASSIGNED_CONTEXT((#11922))
GLOBAL_UNIT_ASSIGNED_CONTEXT((#11934,#11936,#11937))
REPRESENTATION_CONTEXT('','3D')
);
#11934=(
LENGTH_UNIT()
NAMED_UNIT(*)
SI_UNIT(.MILLI.,.METRE.)
);
#11936=(
NAMED_UNIT(*)
PLANE_ANGLE_UNIT()
SI_UNIT($,.RADIAN.)
);
#11937=(
NAMED_UNIT(*)
SI_UNIT($,.STERADIAN.)
SOLID_ANGLE_UNIT()
);
#11945=SHAPE_DEFINITION_REPRESENTATION(#11955,#11994);
#11955=PRODUCT_DEFINITION_SHAPE('',$,#12005);
#11994=SHAPE_REPRESENTATION('',(#7521),#11930);
#11997=PRODUCT_DEFINITION_CONTEXT('part definition',#12029,'design');
#12005=PRODUCT_DEFINITION('Linkage Arm','Linkage Arm',#12015,#11997);
#12015=PRODUCT_DEFINITION_FORMATION('',$,#12038);
#12029=APPLICATION_CONTEXT(
'Core Data for Automotive Mechanical Design Process');
#12030=PRODUCT_CONTEXT('part definition',#12029,'mechanical');
#12038=PRODUCT('Linkage Arm','Linkage Arm',$,(#12030));
#12044=PRESENTATION_STYLE_ASSIGNMENT((#12048));
#12048=SURFACE_STYLE_USAGE(.BOTH.,#12052);
#12052=SURFACE_SIDE_STYLE('',(#12056));
#12056=SURFACE_STYLE_FILL_AREA(#12060);
#12060=FILL_AREA_STYLE('Opaque(97,158,199)',(#12064));
#12064=FILL_AREA_STYLE_COLOUR('Opaque(97,158,199)',#12068);
#12068=COLOUR_RGB('Opaque(97,158,199)',0.380392156862745,0.619607843137255,
0.780392156862745);
ENDSEC;
END-ISO-10303-21;
